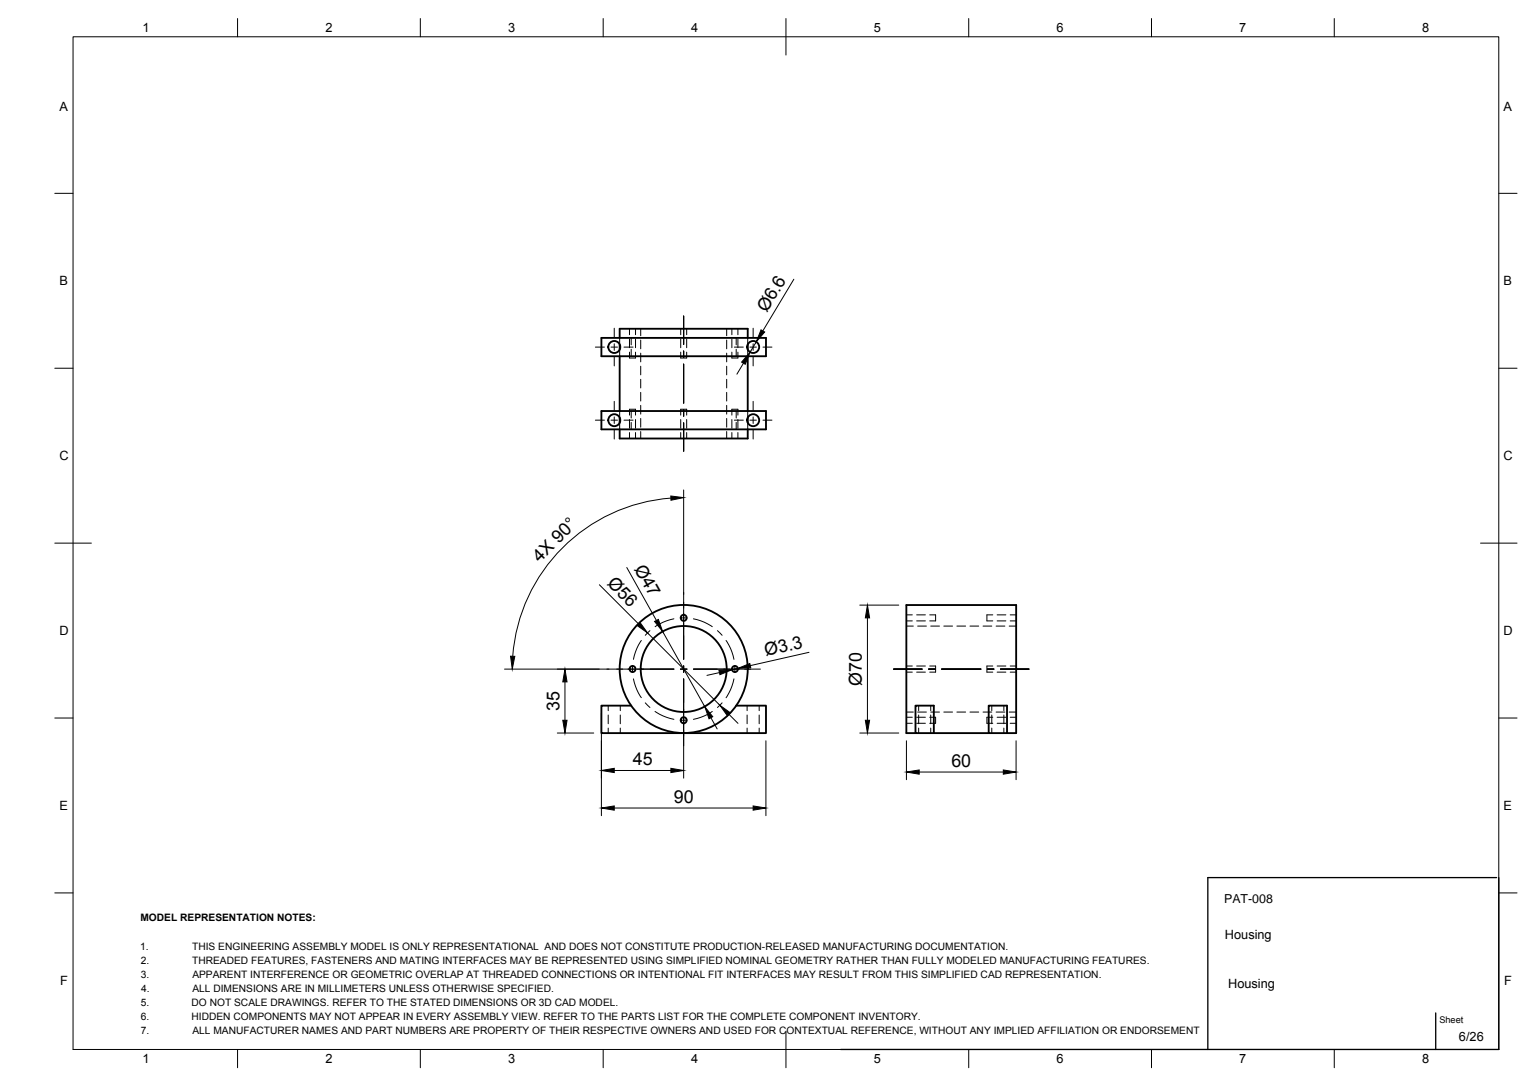
ISO-10303-21;
HEADER;
/* Generated by software containing ST-Developer
 * from STEP Tools, Inc. (www.steptools.com) 
 */

FILE_DESCRIPTION(
/* description */ ('Bearing housing with oil seal and end cap'),
/* implementation_level */ '2;1');

FILE_NAME(
/* name */ 'Housing.step',
/* time_stamp */ '2026-10-28T03:23:10-07:00',
/* author */ (''),
/* organization */ (''),
/* preprocessor_version */ 'ST-DEVELOPER v20.2',
/* originating_system */ 'Autodesk Translation Framework v15.17.0.0',
/* authorisation */ '');

FILE_SCHEMA (('AUTOMOTIVE_DESIGN { 1 0 10303 214 3 1 1 }'));
ENDSEC;

DATA;
#10=MECHANICAL_DESIGN_GEOMETRIC_PRESENTATION_REPRESENTATION('',(#260),#7871);
#218=SHAPE_REPRESENTATION_RELATIONSHIP('SRR','None',#7965,#239);
#239=ADVANCED_BREP_SHAPE_REPRESENTATION('',(#289),#7849);
#260=STYLED_ITEM('',(#8132),#289);
#289=MANIFOLD_SOLID_BREP('Body1',#4086);
#323=FACE_BOUND('',#846,.T.);
#324=FACE_BOUND('',#848,.T.);
#325=FACE_BOUND('',#851,.T.);
#326=FACE_BOUND('',#852,.T.);
#327=FACE_BOUND('',#859,.T.);
#328=FACE_BOUND('',#861,.T.);
#329=FACE_BOUND('',#864,.T.);
#330=FACE_BOUND('',#865,.T.);
#331=FACE_BOUND('',#869,.T.);
#332=FACE_BOUND('',#870,.T.);
#333=FACE_BOUND('',#872,.T.);
#334=FACE_BOUND('',#873,.T.);
#335=FACE_BOUND('',#874,.T.);
#336=FACE_BOUND('',#875,.T.);
#337=FACE_BOUND('',#876,.T.);
#338=FACE_BOUND('',#878,.T.);
#339=FACE_BOUND('',#879,.T.);
#340=FACE_BOUND('',#880,.T.);
#341=FACE_BOUND('',#881,.T.);
#342=FACE_BOUND('',#882,.T.);
#414=PLANE('',#4373);
#415=PLANE('',#4377);
#416=PLANE('',#4381);
#417=PLANE('',#4385);
#418=PLANE('',#4389);
#419=PLANE('',#4393);
#420=PLANE('',#4397);
#421=PLANE('',#4401);
#422=PLANE('',#4414);
#423=PLANE('',#4416);
#424=PLANE('',#4418);
#425=PLANE('',#4420);
#426=PLANE('',#4422);
#427=PLANE('',#4423);
#428=PLANE('',#4424);
#429=PLANE('',#4425);
#430=PLANE('',#4426);
#431=PLANE('',#4427);
#432=PLANE('',#4429);
#433=PLANE('',#4431);
#434=PLANE('',#4433);
#435=PLANE('',#4435);
#436=PLANE('',#4436);
#437=PLANE('',#4437);
#438=PLANE('',#4438);
#439=PLANE('',#4439);
#440=PLANE('',#4446);
#441=PLANE('',#4447);
#562=FACE_OUTER_BOUND('',#821,.T.);
#563=FACE_OUTER_BOUND('',#822,.T.);
#564=FACE_OUTER_BOUND('',#823,.T.);
#565=FACE_OUTER_BOUND('',#824,.T.);
#566=FACE_OUTER_BOUND('',#825,.T.);
#567=FACE_OUTER_BOUND('',#826,.T.);
#568=FACE_OUTER_BOUND('',#827,.T.);
#569=FACE_OUTER_BOUND('',#828,.T.);
#570=FACE_OUTER_BOUND('',#829,.T.);
#571=FACE_OUTER_BOUND('',#830,.T.);
#572=FACE_OUTER_BOUND('',#831,.T.);
#573=FACE_OUTER_BOUND('',#832,.T.);
#574=FACE_OUTER_BOUND('',#833,.T.);
#575=FACE_OUTER_BOUND('',#834,.T.);
#576=FACE_OUTER_BOUND('',#835,.T.);
#577=FACE_OUTER_BOUND('',#836,.T.);
#578=FACE_OUTER_BOUND('',#837,.T.);
#579=FACE_OUTER_BOUND('',#838,.T.);
#580=FACE_OUTER_BOUND('',#839,.T.);
#581=FACE_OUTER_BOUND('',#840,.T.);
#582=FACE_OUTER_BOUND('',#841,.T.);
#583=FACE_OUTER_BOUND('',#842,.T.);
#584=FACE_OUTER_BOUND('',#843,.T.);
#585=FACE_OUTER_BOUND('',#844,.T.);
#586=FACE_OUTER_BOUND('',#845,.T.);
#587=FACE_OUTER_BOUND('',#847,.T.);
#588=FACE_OUTER_BOUND('',#849,.T.);
#589=FACE_OUTER_BOUND('',#850,.T.);
#590=FACE_OUTER_BOUND('',#853,.T.);
#591=FACE_OUTER_BOUND('',#854,.T.);
#592=FACE_OUTER_BOUND('',#855,.T.);
#593=FACE_OUTER_BOUND('',#856,.T.);
#594=FACE_OUTER_BOUND('',#857,.T.);
#595=FACE_OUTER_BOUND('',#858,.T.);
#596=FACE_OUTER_BOUND('',#860,.T.);
#597=FACE_OUTER_BOUND('',#862,.T.);
#598=FACE_OUTER_BOUND('',#863,.T.);
#599=FACE_OUTER_BOUND('',#866,.T.);
#600=FACE_OUTER_BOUND('',#867,.T.);
#601=FACE_OUTER_BOUND('',#868,.T.);
#602=FACE_OUTER_BOUND('',#871,.T.);
#603=FACE_OUTER_BOUND('',#877,.T.);
#821=EDGE_LOOP('',(#2791,#2792,#2793,#2794));
#822=EDGE_LOOP('',(#2795));
#823=EDGE_LOOP('',(#2796,#2797,#2798,#2799));
#824=EDGE_LOOP('',(#2800));
#825=EDGE_LOOP('',(#2801,#2802,#2803,#2804));
#826=EDGE_LOOP('',(#2805));
#827=EDGE_LOOP('',(#2806,#2807,#2808,#2809));
#828=EDGE_LOOP('',(#2810));
#829=EDGE_LOOP('',(#2811,#2812,#2813,#2814));
#830=EDGE_LOOP('',(#2815));
#831=EDGE_LOOP('',(#2816,#2817,#2818,#2819));
#832=EDGE_LOOP('',(#2820));
#833=EDGE_LOOP('',(#2821,#2822,#2823,#2824));
#834=EDGE_LOOP('',(#2825));
#835=EDGE_LOOP('',(#2826,#2827,#2828,#2829));
#836=EDGE_LOOP('',(#2830));
#837=EDGE_LOOP('',(#2831,#2832,#2833,#2834));
#838=EDGE_LOOP('',(#2835,#2836,#2837,#2838));
#839=EDGE_LOOP('',(#2839,#2840,#2841,#2842));
#840=EDGE_LOOP('',(#2843,#2844,#2845,#2846));
#841=EDGE_LOOP('',(#2847,#2848,#2849,#2850));
#842=EDGE_LOOP('',(#2851,#2852,#2853,#2854));
#843=EDGE_LOOP('',(#2855,#2856,#2857,#2858));
#844=EDGE_LOOP('',(#2859,#2860,#2861,#2862));
#845=EDGE_LOOP('',(#2863,#2864,#2865,#2866));
#846=EDGE_LOOP('',(#2867));
#847=EDGE_LOOP('',(#2868,#2869,#2870,#2871));
#848=EDGE_LOOP('',(#2872));
#849=EDGE_LOOP('',(#2873,#2874,#2875,#2876));
#850=EDGE_LOOP('',(#2877,#2878,#2879,#2880,#2881,#2882));
#851=EDGE_LOOP('',(#2883));
#852=EDGE_LOOP('',(#2884));
#853=EDGE_LOOP('',(#2885,#2886,#2887,#2888));
#854=EDGE_LOOP('',(#2889,#2890,#2891,#2892));
#855=EDGE_LOOP('',(#2893,#2894,#2895,#2896));
#856=EDGE_LOOP('',(#2897,#2898,#2899,#2900));
#857=EDGE_LOOP('',(#2901,#2902,#2903,#2904));
#858=EDGE_LOOP('',(#2905,#2906,#2907,#2908));
#859=EDGE_LOOP('',(#2909));
#860=EDGE_LOOP('',(#2910,#2911,#2912,#2913));
#861=EDGE_LOOP('',(#2914));
#862=EDGE_LOOP('',(#2915,#2916,#2917,#2918));
#863=EDGE_LOOP('',(#2919,#2920,#2921,#2922,#2923,#2924));
#864=EDGE_LOOP('',(#2925));
#865=EDGE_LOOP('',(#2926));
#866=EDGE_LOOP('',(#2927,#2928,#2929,#2930));
#867=EDGE_LOOP('',(#2931,#2932,#2933,#2934));
#868=EDGE_LOOP('',(#2935,#2936,#2937,#2938));
#869=EDGE_LOOP('',(#2939,#2940,#2941,#2942,#2943,#2944));
#870=EDGE_LOOP('',(#2945,#2946,#2947,#2948,#2949,#2950));
#871=EDGE_LOOP('',(#2951));
#872=EDGE_LOOP('',(#2952));
#873=EDGE_LOOP('',(#2953));
#874=EDGE_LOOP('',(#2954));
#875=EDGE_LOOP('',(#2955));
#876=EDGE_LOOP('',(#2956));
#877=EDGE_LOOP('',(#2957));
#878=EDGE_LOOP('',(#2958));
#879=EDGE_LOOP('',(#2959));
#880=EDGE_LOOP('',(#2960));
#881=EDGE_LOOP('',(#2961));
#882=EDGE_LOOP('',(#2962));
#1163=LINE('',#6264,#1425);
#1164=LINE('',#6271,#1426);
#1165=LINE('',#6278,#1427);
#1166=LINE('',#6285,#1428);
#1167=LINE('',#6292,#1429);
#1168=LINE('',#6299,#1430);
#1169=LINE('',#6306,#1431);
#1170=LINE('',#6313,#1432);
#1171=LINE('',#6320,#1433);
#1172=LINE('',#6326,#1434);
#1173=LINE('',#6332,#1435);
#1174=LINE('',#6338,#1436);
#1175=LINE('',#6345,#1437);
#1176=LINE('',#6347,#1438);
#1177=LINE('',#6348,#1439);
#1178=LINE('',#6353,#1440);
#1179=LINE('',#6355,#1441);
#1180=LINE('',#6356,#1442);
#1181=LINE('',#6362,#1443);
#1182=LINE('',#6364,#1444);
#1183=LINE('',#6365,#1445);
#1184=LINE('',#6370,#1446);
#1185=LINE('',#6372,#1447);
#1186=LINE('',#6373,#1448);
#1187=LINE('',#6375,#1449);
#1188=LINE('',#6376,#1450);
#1189=LINE('',#6378,#1451);
#1190=LINE('',#6379,#1452);
#1191=LINE('',#6381,#1453);
#1192=LINE('',#6383,#1454);
#1193=LINE('',#6390,#1455);
#1194=LINE('',#6392,#1456);
#1195=LINE('',#6393,#1457);
#1196=LINE('',#6398,#1458);
#1197=LINE('',#6400,#1459);
#1198=LINE('',#6401,#1460);
#1199=LINE('',#6407,#1461);
#1200=LINE('',#6409,#1462);
#1201=LINE('',#6410,#1463);
#1202=LINE('',#6415,#1464);
#1203=LINE('',#6417,#1465);
#1204=LINE('',#6418,#1466);
#1205=LINE('',#6420,#1467);
#1206=LINE('',#6421,#1468);
#1207=LINE('',#6423,#1469);
#1208=LINE('',#6424,#1470);
#1209=LINE('',#6426,#1471);
#1210=LINE('',#6428,#1472);
#1211=LINE('',#6434,#1473);
#1212=LINE('',#6440,#1474);
#1425=VECTOR('',#4944,0.165);
#1426=VECTOR('',#4953,0.165);
#1427=VECTOR('',#4962,0.165);
#1428=VECTOR('',#4971,0.165);
#1429=VECTOR('',#4980,0.165);
#1430=VECTOR('',#4989,0.165);
#1431=VECTOR('',#4998,0.165);
#1432=VECTOR('',#5007,0.165);
#1433=VECTOR('',#5016,0.33);
#1434=VECTOR('',#5023,0.33);
#1435=VECTOR('',#5030,0.33);
#1436=VECTOR('',#5037,0.33);
#1437=VECTOR('',#5044,1.);
#1438=VECTOR('',#5045,1.);
#1439=VECTOR('',#5046,1.);
#1440=VECTOR('',#5051,1.);
#1441=VECTOR('',#5052,1.);
#1442=VECTOR('',#5053,1.);
#1443=VECTOR('',#5058,1.);
#1444=VECTOR('',#5059,1.);
#1445=VECTOR('',#5060,1.);
#1446=VECTOR('',#5065,1.);
#1447=VECTOR('',#5066,1.);
#1448=VECTOR('',#5067,1.);
#1449=VECTOR('',#5070,1.);
#1450=VECTOR('',#5071,1.);
#1451=VECTOR('',#5074,1.);
#1452=VECTOR('',#5075,1.);
#1453=VECTOR('',#5078,1.);
#1454=VECTOR('',#5081,1.);
#1455=VECTOR('',#5088,1.);
#1456=VECTOR('',#5089,1.);
#1457=VECTOR('',#5090,1.);
#1458=VECTOR('',#5095,1.);
#1459=VECTOR('',#5096,1.);
#1460=VECTOR('',#5097,1.);
#1461=VECTOR('',#5102,1.);
#1462=VECTOR('',#5103,1.);
#1463=VECTOR('',#5104,1.);
#1464=VECTOR('',#5109,1.);
#1465=VECTOR('',#5110,1.);
#1466=VECTOR('',#5111,1.);
#1467=VECTOR('',#5114,1.);
#1468=VECTOR('',#5115,1.);
#1469=VECTOR('',#5118,1.);
#1470=VECTOR('',#5119,1.);
#1471=VECTOR('',#5122,1.);
#1472=VECTOR('',#5125,1.);
#1473=VECTOR('',#5132,2.35);
#1474=VECTOR('',#5139,3.5);
#1679=CIRCLE('',#4371,0.165);
#1680=CIRCLE('',#4372,0.165);
#1681=CIRCLE('',#4375,0.165);
#1682=CIRCLE('',#4376,0.165);
#1683=CIRCLE('',#4379,0.165);
#1684=CIRCLE('',#4380,0.165);
#1685=CIRCLE('',#4383,0.165);
#1686=CIRCLE('',#4384,0.165);
#1687=CIRCLE('',#4387,0.165);
#1688=CIRCLE('',#4388,0.165);
#1689=CIRCLE('',#4391,0.165);
#1690=CIRCLE('',#4392,0.165);
#1691=CIRCLE('',#4395,0.165);
#1692=CIRCLE('',#4396,0.165);
#1693=CIRCLE('',#4399,0.165);
#1694=CIRCLE('',#4400,0.165);
#1695=CIRCLE('',#4403,0.33);
#1696=CIRCLE('',#4404,0.33);
#1697=CIRCLE('',#4406,0.33);
#1698=CIRCLE('',#4407,0.33);
#1699=CIRCLE('',#4409,0.33);
#1700=CIRCLE('',#4410,0.33);
#1701=CIRCLE('',#4412,0.33);
#1702=CIRCLE('',#4413,0.33);
#1703=CIRCLE('',#4415,3.5);
#1704=CIRCLE('',#4417,3.5);
#1705=CIRCLE('',#4419,3.5);
#1706=CIRCLE('',#4421,3.5);
#1707=CIRCLE('',#4428,3.5);
#1708=CIRCLE('',#4430,3.5);
#1709=CIRCLE('',#4432,3.5);
#1710=CIRCLE('',#4434,3.5);
#1711=CIRCLE('',#4441,2.35);
#1712=CIRCLE('',#4442,2.35);
#1713=CIRCLE('',#4444,3.5);
#1714=CIRCLE('',#4445,3.5);
#1907=VERTEX_POINT('',#6261);
#1908=VERTEX_POINT('',#6263);
#1909=VERTEX_POINT('',#6268);
#1910=VERTEX_POINT('',#6270);
#1911=VERTEX_POINT('',#6275);
#1912=VERTEX_POINT('',#6277);
#1913=VERTEX_POINT('',#6282);
#1914=VERTEX_POINT('',#6284);
#1915=VERTEX_POINT('',#6289);
#1916=VERTEX_POINT('',#6291);
#1917=VERTEX_POINT('',#6296);
#1918=VERTEX_POINT('',#6298);
#1919=VERTEX_POINT('',#6303);
#1920=VERTEX_POINT('',#6305);
#1921=VERTEX_POINT('',#6310);
#1922=VERTEX_POINT('',#6312);
#1923=VERTEX_POINT('',#6317);
#1924=VERTEX_POINT('',#6319);
#1925=VERTEX_POINT('',#6323);
#1926=VERTEX_POINT('',#6325);
#1927=VERTEX_POINT('',#6329);
#1928=VERTEX_POINT('',#6331);
#1929=VERTEX_POINT('',#6335);
#1930=VERTEX_POINT('',#6337);
#1931=VERTEX_POINT('',#6341);
#1932=VERTEX_POINT('',#6342);
#1933=VERTEX_POINT('',#6344);
#1934=VERTEX_POINT('',#6346);
#1935=VERTEX_POINT('',#6350);
#1936=VERTEX_POINT('',#6352);
#1937=VERTEX_POINT('',#6354);
#1938=VERTEX_POINT('',#6358);
#1939=VERTEX_POINT('',#6359);
#1940=VERTEX_POINT('',#6361);
#1941=VERTEX_POINT('',#6363);
#1942=VERTEX_POINT('',#6367);
#1943=VERTEX_POINT('',#6369);
#1944=VERTEX_POINT('',#6371);
#1945=VERTEX_POINT('',#6386);
#1946=VERTEX_POINT('',#6387);
#1947=VERTEX_POINT('',#6389);
#1948=VERTEX_POINT('',#6391);
#1949=VERTEX_POINT('',#6395);
#1950=VERTEX_POINT('',#6397);
#1951=VERTEX_POINT('',#6399);
#1952=VERTEX_POINT('',#6403);
#1953=VERTEX_POINT('',#6404);
#1954=VERTEX_POINT('',#6406);
#1955=VERTEX_POINT('',#6408);
#1956=VERTEX_POINT('',#6412);
#1957=VERTEX_POINT('',#6414);
#1958=VERTEX_POINT('',#6416);
#1959=VERTEX_POINT('',#6431);
#1960=VERTEX_POINT('',#6433);
#1961=VERTEX_POINT('',#6437);
#1962=VERTEX_POINT('',#6439);
#2259=EDGE_CURVE('',#1907,#1907,#1679,.T.);
#2260=EDGE_CURVE('',#1907,#1908,#1163,.T.);
#2261=EDGE_CURVE('',#1908,#1908,#1680,.T.);
#2262=EDGE_CURVE('',#1909,#1909,#1681,.T.);
#2263=EDGE_CURVE('',#1909,#1910,#1164,.T.);
#2264=EDGE_CURVE('',#1910,#1910,#1682,.T.);
#2265=EDGE_CURVE('',#1911,#1911,#1683,.T.);
#2266=EDGE_CURVE('',#1911,#1912,#1165,.T.);
#2267=EDGE_CURVE('',#1912,#1912,#1684,.T.);
#2268=EDGE_CURVE('',#1913,#1913,#1685,.T.);
#2269=EDGE_CURVE('',#1913,#1914,#1166,.T.);
#2270=EDGE_CURVE('',#1914,#1914,#1686,.T.);
#2271=EDGE_CURVE('',#1915,#1915,#1687,.T.);
#2272=EDGE_CURVE('',#1915,#1916,#1167,.T.);
#2273=EDGE_CURVE('',#1916,#1916,#1688,.T.);
#2274=EDGE_CURVE('',#1917,#1917,#1689,.T.);
#2275=EDGE_CURVE('',#1917,#1918,#1168,.T.);
#2276=EDGE_CURVE('',#1918,#1918,#1690,.T.);
#2277=EDGE_CURVE('',#1919,#1919,#1691,.T.);
#2278=EDGE_CURVE('',#1919,#1920,#1169,.T.);
#2279=EDGE_CURVE('',#1920,#1920,#1692,.T.);
#2280=EDGE_CURVE('',#1921,#1921,#1693,.T.);
#2281=EDGE_CURVE('',#1921,#1922,#1170,.T.);
#2282=EDGE_CURVE('',#1922,#1922,#1694,.T.);
#2283=EDGE_CURVE('',#1923,#1923,#1695,.T.);
#2284=EDGE_CURVE('',#1923,#1924,#1171,.T.);
#2285=EDGE_CURVE('',#1924,#1924,#1696,.T.);
#2286=EDGE_CURVE('',#1925,#1925,#1697,.T.);
#2287=EDGE_CURVE('',#1925,#1926,#1172,.T.);
#2288=EDGE_CURVE('',#1926,#1926,#1698,.T.);
#2289=EDGE_CURVE('',#1927,#1927,#1699,.T.);
#2290=EDGE_CURVE('',#1927,#1928,#1173,.T.);
#2291=EDGE_CURVE('',#1928,#1928,#1700,.T.);
#2292=EDGE_CURVE('',#1929,#1929,#1701,.T.);
#2293=EDGE_CURVE('',#1929,#1930,#1174,.T.);
#2294=EDGE_CURVE('',#1930,#1930,#1702,.T.);
#2295=EDGE_CURVE('',#1931,#1932,#1703,.T.);
#2296=EDGE_CURVE('',#1931,#1933,#1175,.T.);
#2297=EDGE_CURVE('',#1933,#1934,#1176,.T.);
#2298=EDGE_CURVE('',#1934,#1932,#1177,.T.);
#2299=EDGE_CURVE('',#1932,#1935,#1704,.T.);
#2300=EDGE_CURVE('',#1932,#1936,#1178,.T.);
#2301=EDGE_CURVE('',#1936,#1937,#1179,.T.);
#2302=EDGE_CURVE('',#1937,#1935,#1180,.T.);
#2303=EDGE_CURVE('',#1938,#1939,#1705,.T.);
#2304=EDGE_CURVE('',#1938,#1940,#1181,.T.);
#2305=EDGE_CURVE('',#1940,#1941,#1182,.T.);
#2306=EDGE_CURVE('',#1941,#1939,#1183,.T.);
#2307=EDGE_CURVE('',#1942,#1938,#1706,.T.);
#2308=EDGE_CURVE('',#1942,#1943,#1184,.T.);
#2309=EDGE_CURVE('',#1943,#1944,#1185,.T.);
#2310=EDGE_CURVE('',#1944,#1938,#1186,.T.);
#2311=EDGE_CURVE('',#1939,#1931,#1187,.T.);
#2312=EDGE_CURVE('',#1941,#1933,#1188,.T.);
#2313=EDGE_CURVE('',#1935,#1942,#1189,.T.);
#2314=EDGE_CURVE('',#1943,#1937,#1190,.T.);
#2315=EDGE_CURVE('',#1944,#1936,#1191,.T.);
#2316=EDGE_CURVE('',#1940,#1934,#1192,.T.);
#2317=EDGE_CURVE('',#1945,#1946,#1707,.T.);
#2318=EDGE_CURVE('',#1945,#1947,#1193,.T.);
#2319=EDGE_CURVE('',#1947,#1948,#1194,.T.);
#2320=EDGE_CURVE('',#1948,#1946,#1195,.T.);
#2321=EDGE_CURVE('',#1946,#1949,#1708,.T.);
#2322=EDGE_CURVE('',#1946,#1950,#1196,.T.);
#2323=EDGE_CURVE('',#1950,#1951,#1197,.T.);
#2324=EDGE_CURVE('',#1951,#1949,#1198,.T.);
#2325=EDGE_CURVE('',#1952,#1953,#1709,.T.);
#2326=EDGE_CURVE('',#1952,#1954,#1199,.T.);
#2327=EDGE_CURVE('',#1954,#1955,#1200,.T.);
#2328=EDGE_CURVE('',#1955,#1953,#1201,.T.);
#2329=EDGE_CURVE('',#1956,#1952,#1710,.T.);
#2330=EDGE_CURVE('',#1956,#1957,#1202,.T.);
#2331=EDGE_CURVE('',#1957,#1958,#1203,.T.);
#2332=EDGE_CURVE('',#1958,#1952,#1204,.T.);
#2333=EDGE_CURVE('',#1953,#1945,#1205,.T.);
#2334=EDGE_CURVE('',#1955,#1947,#1206,.T.);
#2335=EDGE_CURVE('',#1949,#1956,#1207,.T.);
#2336=EDGE_CURVE('',#1957,#1951,#1208,.T.);
#2337=EDGE_CURVE('',#1958,#1950,#1209,.T.);
#2338=EDGE_CURVE('',#1954,#1948,#1210,.T.);
#2339=EDGE_CURVE('',#1959,#1959,#1711,.T.);
#2340=EDGE_CURVE('',#1959,#1960,#1211,.T.);
#2341=EDGE_CURVE('',#1960,#1960,#1712,.T.);
#2342=EDGE_CURVE('',#1961,#1961,#1713,.T.);
#2343=EDGE_CURVE('',#1961,#1962,#1212,.T.);
#2344=EDGE_CURVE('',#1962,#1962,#1714,.T.);
#2791=ORIENTED_EDGE('',*,*,#2259,.F.);
#2792=ORIENTED_EDGE('',*,*,#2260,.T.);
#2793=ORIENTED_EDGE('',*,*,#2261,.F.);
#2794=ORIENTED_EDGE('',*,*,#2260,.F.);
#2795=ORIENTED_EDGE('',*,*,#2259,.T.);
#2796=ORIENTED_EDGE('',*,*,#2262,.F.);
#2797=ORIENTED_EDGE('',*,*,#2263,.T.);
#2798=ORIENTED_EDGE('',*,*,#2264,.F.);
#2799=ORIENTED_EDGE('',*,*,#2263,.F.);
#2800=ORIENTED_EDGE('',*,*,#2262,.T.);
#2801=ORIENTED_EDGE('',*,*,#2265,.F.);
#2802=ORIENTED_EDGE('',*,*,#2266,.T.);
#2803=ORIENTED_EDGE('',*,*,#2267,.F.);
#2804=ORIENTED_EDGE('',*,*,#2266,.F.);
#2805=ORIENTED_EDGE('',*,*,#2265,.T.);
#2806=ORIENTED_EDGE('',*,*,#2268,.F.);
#2807=ORIENTED_EDGE('',*,*,#2269,.T.);
#2808=ORIENTED_EDGE('',*,*,#2270,.F.);
#2809=ORIENTED_EDGE('',*,*,#2269,.F.);
#2810=ORIENTED_EDGE('',*,*,#2268,.T.);
#2811=ORIENTED_EDGE('',*,*,#2271,.F.);
#2812=ORIENTED_EDGE('',*,*,#2272,.T.);
#2813=ORIENTED_EDGE('',*,*,#2273,.T.);
#2814=ORIENTED_EDGE('',*,*,#2272,.F.);
#2815=ORIENTED_EDGE('',*,*,#2273,.F.);
#2816=ORIENTED_EDGE('',*,*,#2274,.F.);
#2817=ORIENTED_EDGE('',*,*,#2275,.T.);
#2818=ORIENTED_EDGE('',*,*,#2276,.T.);
#2819=ORIENTED_EDGE('',*,*,#2275,.F.);
#2820=ORIENTED_EDGE('',*,*,#2276,.F.);
#2821=ORIENTED_EDGE('',*,*,#2277,.F.);
#2822=ORIENTED_EDGE('',*,*,#2278,.T.);
#2823=ORIENTED_EDGE('',*,*,#2279,.T.);
#2824=ORIENTED_EDGE('',*,*,#2278,.F.);
#2825=ORIENTED_EDGE('',*,*,#2279,.F.);
#2826=ORIENTED_EDGE('',*,*,#2280,.F.);
#2827=ORIENTED_EDGE('',*,*,#2281,.T.);
#2828=ORIENTED_EDGE('',*,*,#2282,.T.);
#2829=ORIENTED_EDGE('',*,*,#2281,.F.);
#2830=ORIENTED_EDGE('',*,*,#2282,.F.);
#2831=ORIENTED_EDGE('',*,*,#2283,.F.);
#2832=ORIENTED_EDGE('',*,*,#2284,.T.);
#2833=ORIENTED_EDGE('',*,*,#2285,.F.);
#2834=ORIENTED_EDGE('',*,*,#2284,.F.);
#2835=ORIENTED_EDGE('',*,*,#2286,.F.);
#2836=ORIENTED_EDGE('',*,*,#2287,.T.);
#2837=ORIENTED_EDGE('',*,*,#2288,.F.);
#2838=ORIENTED_EDGE('',*,*,#2287,.F.);
#2839=ORIENTED_EDGE('',*,*,#2289,.F.);
#2840=ORIENTED_EDGE('',*,*,#2290,.T.);
#2841=ORIENTED_EDGE('',*,*,#2291,.F.);
#2842=ORIENTED_EDGE('',*,*,#2290,.F.);
#2843=ORIENTED_EDGE('',*,*,#2292,.F.);
#2844=ORIENTED_EDGE('',*,*,#2293,.T.);
#2845=ORIENTED_EDGE('',*,*,#2294,.F.);
#2846=ORIENTED_EDGE('',*,*,#2293,.F.);
#2847=ORIENTED_EDGE('',*,*,#2295,.F.);
#2848=ORIENTED_EDGE('',*,*,#2296,.T.);
#2849=ORIENTED_EDGE('',*,*,#2297,.T.);
#2850=ORIENTED_EDGE('',*,*,#2298,.T.);
#2851=ORIENTED_EDGE('',*,*,#2299,.F.);
#2852=ORIENTED_EDGE('',*,*,#2300,.T.);
#2853=ORIENTED_EDGE('',*,*,#2301,.T.);
#2854=ORIENTED_EDGE('',*,*,#2302,.T.);
#2855=ORIENTED_EDGE('',*,*,#2303,.F.);
#2856=ORIENTED_EDGE('',*,*,#2304,.T.);
#2857=ORIENTED_EDGE('',*,*,#2305,.T.);
#2858=ORIENTED_EDGE('',*,*,#2306,.T.);
#2859=ORIENTED_EDGE('',*,*,#2307,.F.);
#2860=ORIENTED_EDGE('',*,*,#2308,.T.);
#2861=ORIENTED_EDGE('',*,*,#2309,.T.);
#2862=ORIENTED_EDGE('',*,*,#2310,.T.);
#2863=ORIENTED_EDGE('',*,*,#2311,.F.);
#2864=ORIENTED_EDGE('',*,*,#2306,.F.);
#2865=ORIENTED_EDGE('',*,*,#2312,.T.);
#2866=ORIENTED_EDGE('',*,*,#2296,.F.);
#2867=ORIENTED_EDGE('',*,*,#2294,.T.);
#2868=ORIENTED_EDGE('',*,*,#2313,.F.);
#2869=ORIENTED_EDGE('',*,*,#2302,.F.);
#2870=ORIENTED_EDGE('',*,*,#2314,.F.);
#2871=ORIENTED_EDGE('',*,*,#2308,.F.);
#2872=ORIENTED_EDGE('',*,*,#2288,.T.);
#2873=ORIENTED_EDGE('',*,*,#2309,.F.);
#2874=ORIENTED_EDGE('',*,*,#2314,.T.);
#2875=ORIENTED_EDGE('',*,*,#2301,.F.);
#2876=ORIENTED_EDGE('',*,*,#2315,.F.);
#2877=ORIENTED_EDGE('',*,*,#2298,.F.);
#2878=ORIENTED_EDGE('',*,*,#2316,.F.);
#2879=ORIENTED_EDGE('',*,*,#2304,.F.);
#2880=ORIENTED_EDGE('',*,*,#2310,.F.);
#2881=ORIENTED_EDGE('',*,*,#2315,.T.);
#2882=ORIENTED_EDGE('',*,*,#2300,.F.);
#2883=ORIENTED_EDGE('',*,*,#2286,.T.);
#2884=ORIENTED_EDGE('',*,*,#2292,.T.);
#2885=ORIENTED_EDGE('',*,*,#2305,.F.);
#2886=ORIENTED_EDGE('',*,*,#2316,.T.);
#2887=ORIENTED_EDGE('',*,*,#2297,.F.);
#2888=ORIENTED_EDGE('',*,*,#2312,.F.);
#2889=ORIENTED_EDGE('',*,*,#2317,.F.);
#2890=ORIENTED_EDGE('',*,*,#2318,.T.);
#2891=ORIENTED_EDGE('',*,*,#2319,.T.);
#2892=ORIENTED_EDGE('',*,*,#2320,.T.);
#2893=ORIENTED_EDGE('',*,*,#2321,.F.);
#2894=ORIENTED_EDGE('',*,*,#2322,.T.);
#2895=ORIENTED_EDGE('',*,*,#2323,.T.);
#2896=ORIENTED_EDGE('',*,*,#2324,.T.);
#2897=ORIENTED_EDGE('',*,*,#2325,.F.);
#2898=ORIENTED_EDGE('',*,*,#2326,.T.);
#2899=ORIENTED_EDGE('',*,*,#2327,.T.);
#2900=ORIENTED_EDGE('',*,*,#2328,.T.);
#2901=ORIENTED_EDGE('',*,*,#2329,.F.);
#2902=ORIENTED_EDGE('',*,*,#2330,.T.);
#2903=ORIENTED_EDGE('',*,*,#2331,.T.);
#2904=ORIENTED_EDGE('',*,*,#2332,.T.);
#2905=ORIENTED_EDGE('',*,*,#2333,.F.);
#2906=ORIENTED_EDGE('',*,*,#2328,.F.);
#2907=ORIENTED_EDGE('',*,*,#2334,.T.);
#2908=ORIENTED_EDGE('',*,*,#2318,.F.);
#2909=ORIENTED_EDGE('',*,*,#2285,.T.);
#2910=ORIENTED_EDGE('',*,*,#2335,.F.);
#2911=ORIENTED_EDGE('',*,*,#2324,.F.);
#2912=ORIENTED_EDGE('',*,*,#2336,.F.);
#2913=ORIENTED_EDGE('',*,*,#2330,.F.);
#2914=ORIENTED_EDGE('',*,*,#2291,.T.);
#2915=ORIENTED_EDGE('',*,*,#2331,.F.);
#2916=ORIENTED_EDGE('',*,*,#2336,.T.);
#2917=ORIENTED_EDGE('',*,*,#2323,.F.);
#2918=ORIENTED_EDGE('',*,*,#2337,.F.);
#2919=ORIENTED_EDGE('',*,*,#2320,.F.);
#2920=ORIENTED_EDGE('',*,*,#2338,.F.);
#2921=ORIENTED_EDGE('',*,*,#2326,.F.);
#2922=ORIENTED_EDGE('',*,*,#2332,.F.);
#2923=ORIENTED_EDGE('',*,*,#2337,.T.);
#2924=ORIENTED_EDGE('',*,*,#2322,.F.);
#2925=ORIENTED_EDGE('',*,*,#2283,.T.);
#2926=ORIENTED_EDGE('',*,*,#2289,.T.);
#2927=ORIENTED_EDGE('',*,*,#2327,.F.);
#2928=ORIENTED_EDGE('',*,*,#2338,.T.);
#2929=ORIENTED_EDGE('',*,*,#2319,.F.);
#2930=ORIENTED_EDGE('',*,*,#2334,.F.);
#2931=ORIENTED_EDGE('',*,*,#2339,.F.);
#2932=ORIENTED_EDGE('',*,*,#2340,.T.);
#2933=ORIENTED_EDGE('',*,*,#2341,.T.);
#2934=ORIENTED_EDGE('',*,*,#2340,.F.);
#2935=ORIENTED_EDGE('',*,*,#2342,.F.);
#2936=ORIENTED_EDGE('',*,*,#2343,.T.);
#2937=ORIENTED_EDGE('',*,*,#2344,.T.);
#2938=ORIENTED_EDGE('',*,*,#2343,.F.);
#2939=ORIENTED_EDGE('',*,*,#2311,.T.);
#2940=ORIENTED_EDGE('',*,*,#2295,.T.);
#2941=ORIENTED_EDGE('',*,*,#2299,.T.);
#2942=ORIENTED_EDGE('',*,*,#2313,.T.);
#2943=ORIENTED_EDGE('',*,*,#2307,.T.);
#2944=ORIENTED_EDGE('',*,*,#2303,.T.);
#2945=ORIENTED_EDGE('',*,*,#2333,.T.);
#2946=ORIENTED_EDGE('',*,*,#2317,.T.);
#2947=ORIENTED_EDGE('',*,*,#2321,.T.);
#2948=ORIENTED_EDGE('',*,*,#2335,.T.);
#2949=ORIENTED_EDGE('',*,*,#2329,.T.);
#2950=ORIENTED_EDGE('',*,*,#2325,.T.);
#2951=ORIENTED_EDGE('',*,*,#2342,.T.);
#2952=ORIENTED_EDGE('',*,*,#2339,.T.);
#2953=ORIENTED_EDGE('',*,*,#2270,.T.);
#2954=ORIENTED_EDGE('',*,*,#2267,.T.);
#2955=ORIENTED_EDGE('',*,*,#2264,.T.);
#2956=ORIENTED_EDGE('',*,*,#2261,.T.);
#2957=ORIENTED_EDGE('',*,*,#2344,.F.);
#2958=ORIENTED_EDGE('',*,*,#2341,.F.);
#2959=ORIENTED_EDGE('',*,*,#2280,.T.);
#2960=ORIENTED_EDGE('',*,*,#2277,.T.);
#2961=ORIENTED_EDGE('',*,*,#2274,.T.);
#2962=ORIENTED_EDGE('',*,*,#2271,.T.);
#3763=CYLINDRICAL_SURFACE('',#4370,0.165);
#3764=CYLINDRICAL_SURFACE('',#4374,0.165);
#3765=CYLINDRICAL_SURFACE('',#4378,0.165);
#3766=CYLINDRICAL_SURFACE('',#4382,0.165);
#3767=CYLINDRICAL_SURFACE('',#4386,0.165);
#3768=CYLINDRICAL_SURFACE('',#4390,0.165);
#3769=CYLINDRICAL_SURFACE('',#4394,0.165);
#3770=CYLINDRICAL_SURFACE('',#4398,0.165);
#3771=CYLINDRICAL_SURFACE('',#4402,0.33);
#3772=CYLINDRICAL_SURFACE('',#4405,0.33);
#3773=CYLINDRICAL_SURFACE('',#4408,0.33);
#3774=CYLINDRICAL_SURFACE('',#4411,0.33);
#3775=CYLINDRICAL_SURFACE('',#4440,2.35);
#3776=CYLINDRICAL_SURFACE('',#4443,3.5);
#3844=ADVANCED_FACE('',(#562),#3763,.F.);
#3845=ADVANCED_FACE('',(#563),#414,.T.);
#3846=ADVANCED_FACE('',(#564),#3764,.F.);
#3847=ADVANCED_FACE('',(#565),#415,.T.);
#3848=ADVANCED_FACE('',(#566),#3765,.F.);
#3849=ADVANCED_FACE('',(#567),#416,.T.);
#3850=ADVANCED_FACE('',(#568),#3766,.F.);
#3851=ADVANCED_FACE('',(#569),#417,.T.);
#3852=ADVANCED_FACE('',(#570),#3767,.F.);
#3853=ADVANCED_FACE('',(#571),#418,.F.);
#3854=ADVANCED_FACE('',(#572),#3768,.F.);
#3855=ADVANCED_FACE('',(#573),#419,.F.);
#3856=ADVANCED_FACE('',(#574),#3769,.F.);
#3857=ADVANCED_FACE('',(#575),#420,.F.);
#3858=ADVANCED_FACE('',(#576),#3770,.F.);
#3859=ADVANCED_FACE('',(#577),#421,.F.);
#3860=ADVANCED_FACE('',(#578),#3771,.F.);
#3861=ADVANCED_FACE('',(#579),#3772,.F.);
#3862=ADVANCED_FACE('',(#580),#3773,.F.);
#3863=ADVANCED_FACE('',(#581),#3774,.F.);
#3864=ADVANCED_FACE('',(#582),#422,.T.);
#3865=ADVANCED_FACE('',(#583),#423,.T.);
#3866=ADVANCED_FACE('',(#584),#424,.F.);
#3867=ADVANCED_FACE('',(#585),#425,.F.);
#3868=ADVANCED_FACE('',(#586,#323),#426,.T.);
#3869=ADVANCED_FACE('',(#587,#324),#427,.T.);
#3870=ADVANCED_FACE('',(#588),#428,.T.);
#3871=ADVANCED_FACE('',(#589,#325,#326),#429,.T.);
#3872=ADVANCED_FACE('',(#590),#430,.T.);
#3873=ADVANCED_FACE('',(#591),#431,.T.);
#3874=ADVANCED_FACE('',(#592),#432,.T.);
#3875=ADVANCED_FACE('',(#593),#433,.F.);
#3876=ADVANCED_FACE('',(#594),#434,.F.);
#3877=ADVANCED_FACE('',(#595,#327),#435,.T.);
#3878=ADVANCED_FACE('',(#596,#328),#436,.T.);
#3879=ADVANCED_FACE('',(#597),#437,.T.);
#3880=ADVANCED_FACE('',(#598,#329,#330),#438,.T.);
#3881=ADVANCED_FACE('',(#599),#439,.T.);
#3882=ADVANCED_FACE('',(#600),#3775,.F.);
#3883=ADVANCED_FACE('',(#601,#331,#332),#3776,.T.);
#3884=ADVANCED_FACE('',(#602,#333,#334,#335,#336,#337),#440,.T.);
#3885=ADVANCED_FACE('',(#603,#338,#339,#340,#341,#342),#441,.F.);
#4086=CLOSED_SHELL('',(#3844,#3845,#3846,#3847,#3848,#3849,#3850,#3851,
#3852,#3853,#3854,#3855,#3856,#3857,#3858,#3859,#3860,#3861,#3862,#3863,
#3864,#3865,#3866,#3867,#3868,#3869,#3870,#3871,#3872,#3873,#3874,#3875,
#3876,#3877,#3878,#3879,#3880,#3881,#3882,#3883,#3884,#3885));
#4369=AXIS2_PLACEMENT_3D('',#6259,#4938,#4939);
#4370=AXIS2_PLACEMENT_3D('',#6260,#4940,#4941);
#4371=AXIS2_PLACEMENT_3D('',#6262,#4942,#4943);
#4372=AXIS2_PLACEMENT_3D('',#6265,#4945,#4946);
#4373=AXIS2_PLACEMENT_3D('',#6266,#4947,#4948);
#4374=AXIS2_PLACEMENT_3D('',#6267,#4949,#4950);
#4375=AXIS2_PLACEMENT_3D('',#6269,#4951,#4952);
#4376=AXIS2_PLACEMENT_3D('',#6272,#4954,#4955);
#4377=AXIS2_PLACEMENT_3D('',#6273,#4956,#4957);
#4378=AXIS2_PLACEMENT_3D('',#6274,#4958,#4959);
#4379=AXIS2_PLACEMENT_3D('',#6276,#4960,#4961);
#4380=AXIS2_PLACEMENT_3D('',#6279,#4963,#4964);
#4381=AXIS2_PLACEMENT_3D('',#6280,#4965,#4966);
#4382=AXIS2_PLACEMENT_3D('',#6281,#4967,#4968);
#4383=AXIS2_PLACEMENT_3D('',#6283,#4969,#4970);
#4384=AXIS2_PLACEMENT_3D('',#6286,#4972,#4973);
#4385=AXIS2_PLACEMENT_3D('',#6287,#4974,#4975);
#4386=AXIS2_PLACEMENT_3D('',#6288,#4976,#4977);
#4387=AXIS2_PLACEMENT_3D('',#6290,#4978,#4979);
#4388=AXIS2_PLACEMENT_3D('',#6293,#4981,#4982);
#4389=AXIS2_PLACEMENT_3D('',#6294,#4983,#4984);
#4390=AXIS2_PLACEMENT_3D('',#6295,#4985,#4986);
#4391=AXIS2_PLACEMENT_3D('',#6297,#4987,#4988);
#4392=AXIS2_PLACEMENT_3D('',#6300,#4990,#4991);
#4393=AXIS2_PLACEMENT_3D('',#6301,#4992,#4993);
#4394=AXIS2_PLACEMENT_3D('',#6302,#4994,#4995);
#4395=AXIS2_PLACEMENT_3D('',#6304,#4996,#4997);
#4396=AXIS2_PLACEMENT_3D('',#6307,#4999,#5000);
#4397=AXIS2_PLACEMENT_3D('',#6308,#5001,#5002);
#4398=AXIS2_PLACEMENT_3D('',#6309,#5003,#5004);
#4399=AXIS2_PLACEMENT_3D('',#6311,#5005,#5006);
#4400=AXIS2_PLACEMENT_3D('',#6314,#5008,#5009);
#4401=AXIS2_PLACEMENT_3D('',#6315,#5010,#5011);
#4402=AXIS2_PLACEMENT_3D('',#6316,#5012,#5013);
#4403=AXIS2_PLACEMENT_3D('',#6318,#5014,#5015);
#4404=AXIS2_PLACEMENT_3D('',#6321,#5017,#5018);
#4405=AXIS2_PLACEMENT_3D('',#6322,#5019,#5020);
#4406=AXIS2_PLACEMENT_3D('',#6324,#5021,#5022);
#4407=AXIS2_PLACEMENT_3D('',#6327,#5024,#5025);
#4408=AXIS2_PLACEMENT_3D('',#6328,#5026,#5027);
#4409=AXIS2_PLACEMENT_3D('',#6330,#5028,#5029);
#4410=AXIS2_PLACEMENT_3D('',#6333,#5031,#5032);
#4411=AXIS2_PLACEMENT_3D('',#6334,#5033,#5034);
#4412=AXIS2_PLACEMENT_3D('',#6336,#5035,#5036);
#4413=AXIS2_PLACEMENT_3D('',#6339,#5038,#5039);
#4414=AXIS2_PLACEMENT_3D('',#6340,#5040,#5041);
#4415=AXIS2_PLACEMENT_3D('',#6343,#5042,#5043);
#4416=AXIS2_PLACEMENT_3D('',#6349,#5047,#5048);
#4417=AXIS2_PLACEMENT_3D('',#6351,#5049,#5050);
#4418=AXIS2_PLACEMENT_3D('',#6357,#5054,#5055);
#4419=AXIS2_PLACEMENT_3D('',#6360,#5056,#5057);
#4420=AXIS2_PLACEMENT_3D('',#6366,#5061,#5062);
#4421=AXIS2_PLACEMENT_3D('',#6368,#5063,#5064);
#4422=AXIS2_PLACEMENT_3D('',#6374,#5068,#5069);
#4423=AXIS2_PLACEMENT_3D('',#6377,#5072,#5073);
#4424=AXIS2_PLACEMENT_3D('',#6380,#5076,#5077);
#4425=AXIS2_PLACEMENT_3D('',#6382,#5079,#5080);
#4426=AXIS2_PLACEMENT_3D('',#6384,#5082,#5083);
#4427=AXIS2_PLACEMENT_3D('',#6385,#5084,#5085);
#4428=AXIS2_PLACEMENT_3D('',#6388,#5086,#5087);
#4429=AXIS2_PLACEMENT_3D('',#6394,#5091,#5092);
#4430=AXIS2_PLACEMENT_3D('',#6396,#5093,#5094);
#4431=AXIS2_PLACEMENT_3D('',#6402,#5098,#5099);
#4432=AXIS2_PLACEMENT_3D('',#6405,#5100,#5101);
#4433=AXIS2_PLACEMENT_3D('',#6411,#5105,#5106);
#4434=AXIS2_PLACEMENT_3D('',#6413,#5107,#5108);
#4435=AXIS2_PLACEMENT_3D('',#6419,#5112,#5113);
#4436=AXIS2_PLACEMENT_3D('',#6422,#5116,#5117);
#4437=AXIS2_PLACEMENT_3D('',#6425,#5120,#5121);
#4438=AXIS2_PLACEMENT_3D('',#6427,#5123,#5124);
#4439=AXIS2_PLACEMENT_3D('',#6429,#5126,#5127);
#4440=AXIS2_PLACEMENT_3D('',#6430,#5128,#5129);
#4441=AXIS2_PLACEMENT_3D('',#6432,#5130,#5131);
#4442=AXIS2_PLACEMENT_3D('',#6435,#5133,#5134);
#4443=AXIS2_PLACEMENT_3D('',#6436,#5135,#5136);
#4444=AXIS2_PLACEMENT_3D('',#6438,#5137,#5138);
#4445=AXIS2_PLACEMENT_3D('',#6441,#5140,#5141);
#4446=AXIS2_PLACEMENT_3D('',#6442,#5142,#5143);
#4447=AXIS2_PLACEMENT_3D('',#6443,#5144,#5145);
#4938=DIRECTION('axis',(0.,0.,1.));
#4939=DIRECTION('refdir',(1.,0.,0.));
#4940=DIRECTION('center_axis',(0.,1.,0.));
#4941=DIRECTION('ref_axis',(1.,0.,0.));
#4942=DIRECTION('center_axis',(0.,1.,0.));
#4943=DIRECTION('ref_axis',(1.,0.,0.));
#4944=DIRECTION('',(0.,1.,0.));
#4945=DIRECTION('center_axis',(0.,-1.,0.));
#4946=DIRECTION('ref_axis',(1.,0.,0.));
#4947=DIRECTION('center_axis',(0.,1.,0.));
#4948=DIRECTION('ref_axis',(1.,0.,0.));
#4949=DIRECTION('center_axis',(0.,1.,0.));
#4950=DIRECTION('ref_axis',(1.,0.,0.));
#4951=DIRECTION('center_axis',(0.,1.,0.));
#4952=DIRECTION('ref_axis',(1.,0.,0.));
#4953=DIRECTION('',(0.,1.,0.));
#4954=DIRECTION('center_axis',(0.,-1.,0.));
#4955=DIRECTION('ref_axis',(1.,0.,0.));
#4956=DIRECTION('center_axis',(0.,1.,0.));
#4957=DIRECTION('ref_axis',(1.,0.,0.));
#4958=DIRECTION('center_axis',(0.,1.,0.));
#4959=DIRECTION('ref_axis',(1.,0.,0.));
#4960=DIRECTION('center_axis',(0.,1.,0.));
#4961=DIRECTION('ref_axis',(1.,0.,0.));
#4962=DIRECTION('',(0.,1.,0.));
#4963=DIRECTION('center_axis',(0.,-1.,0.));
#4964=DIRECTION('ref_axis',(1.,0.,0.));
#4965=DIRECTION('center_axis',(0.,1.,0.));
#4966=DIRECTION('ref_axis',(1.,0.,0.));
#4967=DIRECTION('center_axis',(0.,1.,0.));
#4968=DIRECTION('ref_axis',(1.,0.,0.));
#4969=DIRECTION('center_axis',(0.,1.,0.));
#4970=DIRECTION('ref_axis',(1.,0.,0.));
#4971=DIRECTION('',(0.,1.,0.));
#4972=DIRECTION('center_axis',(0.,-1.,0.));
#4973=DIRECTION('ref_axis',(1.,0.,0.));
#4974=DIRECTION('center_axis',(0.,1.,0.));
#4975=DIRECTION('ref_axis',(1.,0.,0.));
#4976=DIRECTION('center_axis',(0.,1.,0.));
#4977=DIRECTION('ref_axis',(1.,0.,0.));
#4978=DIRECTION('center_axis',(0.,1.,0.));
#4979=DIRECTION('ref_axis',(1.,0.,0.));
#4980=DIRECTION('',(0.,1.,0.));
#4981=DIRECTION('center_axis',(0.,1.,0.));
#4982=DIRECTION('ref_axis',(1.,0.,0.));
#4983=DIRECTION('center_axis',(0.,1.,0.));
#4984=DIRECTION('ref_axis',(1.,0.,0.));
#4985=DIRECTION('center_axis',(0.,1.,0.));
#4986=DIRECTION('ref_axis',(1.,0.,0.));
#4987=DIRECTION('center_axis',(0.,1.,0.));
#4988=DIRECTION('ref_axis',(1.,0.,0.));
#4989=DIRECTION('',(0.,1.,0.));
#4990=DIRECTION('center_axis',(0.,1.,0.));
#4991=DIRECTION('ref_axis',(1.,0.,0.));
#4992=DIRECTION('center_axis',(0.,1.,0.));
#4993=DIRECTION('ref_axis',(1.,0.,0.));
#4994=DIRECTION('center_axis',(0.,1.,0.));
#4995=DIRECTION('ref_axis',(1.,0.,0.));
#4996=DIRECTION('center_axis',(0.,1.,0.));
#4997=DIRECTION('ref_axis',(1.,0.,0.));
#4998=DIRECTION('',(0.,1.,0.));
#4999=DIRECTION('center_axis',(0.,1.,0.));
#5000=DIRECTION('ref_axis',(1.,0.,0.));
#5001=DIRECTION('center_axis',(0.,1.,0.));
#5002=DIRECTION('ref_axis',(1.,0.,0.));
#5003=DIRECTION('center_axis',(0.,1.,0.));
#5004=DIRECTION('ref_axis',(1.,0.,0.));
#5005=DIRECTION('center_axis',(0.,1.,0.));
#5006=DIRECTION('ref_axis',(1.,0.,0.));
#5007=DIRECTION('',(0.,1.,0.));
#5008=DIRECTION('center_axis',(0.,1.,0.));
#5009=DIRECTION('ref_axis',(1.,0.,0.));
#5010=DIRECTION('center_axis',(0.,1.,0.));
#5011=DIRECTION('ref_axis',(1.,0.,0.));
#5012=DIRECTION('center_axis',(0.,0.,1.));
#5013=DIRECTION('ref_axis',(1.,0.,0.));
#5014=DIRECTION('center_axis',(0.,0.,1.));
#5015=DIRECTION('ref_axis',(1.,0.,0.));
#5016=DIRECTION('',(0.,0.,1.));
#5017=DIRECTION('center_axis',(0.,0.,-1.));
#5018=DIRECTION('ref_axis',(1.,0.,0.));
#5019=DIRECTION('center_axis',(0.,0.,1.));
#5020=DIRECTION('ref_axis',(1.,0.,0.));
#5021=DIRECTION('center_axis',(0.,0.,1.));
#5022=DIRECTION('ref_axis',(1.,0.,0.));
#5023=DIRECTION('',(0.,0.,1.));
#5024=DIRECTION('center_axis',(0.,0.,-1.));
#5025=DIRECTION('ref_axis',(1.,0.,0.));
#5026=DIRECTION('center_axis',(0.,0.,1.));
#5027=DIRECTION('ref_axis',(1.,0.,0.));
#5028=DIRECTION('center_axis',(0.,0.,1.));
#5029=DIRECTION('ref_axis',(1.,0.,0.));
#5030=DIRECTION('',(0.,0.,1.));
#5031=DIRECTION('center_axis',(0.,0.,-1.));
#5032=DIRECTION('ref_axis',(1.,0.,0.));
#5033=DIRECTION('center_axis',(0.,0.,1.));
#5034=DIRECTION('ref_axis',(1.,0.,0.));
#5035=DIRECTION('center_axis',(0.,0.,1.));
#5036=DIRECTION('ref_axis',(1.,0.,0.));
#5037=DIRECTION('',(0.,0.,1.));
#5038=DIRECTION('center_axis',(0.,0.,-1.));
#5039=DIRECTION('ref_axis',(1.,0.,0.));
#5040=DIRECTION('center_axis',(0.,1.,0.));
#5041=DIRECTION('ref_axis',(0.,0.,1.));
#5042=DIRECTION('center_axis',(0.,1.,0.));
#5043=DIRECTION('ref_axis',(1.,0.,0.));
#5044=DIRECTION('',(1.,0.,0.));
#5045=DIRECTION('',(0.,0.,-1.));
#5046=DIRECTION('',(-1.,0.,0.));
#5047=DIRECTION('center_axis',(0.,1.,0.));
#5048=DIRECTION('ref_axis',(0.,0.,1.));
#5049=DIRECTION('center_axis',(0.,1.,0.));
#5050=DIRECTION('ref_axis',(1.,0.,0.));
#5051=DIRECTION('',(-1.,0.,0.));
#5052=DIRECTION('',(0.,0.,1.));
#5053=DIRECTION('',(1.,0.,0.));
#5054=DIRECTION('center_axis',(0.,1.,0.));
#5055=DIRECTION('ref_axis',(1.,0.,0.));
#5056=DIRECTION('center_axis',(0.,-1.,0.));
#5057=DIRECTION('ref_axis',(1.,0.,0.));
#5058=DIRECTION('',(1.,0.,0.));
#5059=DIRECTION('',(0.,0.,1.));
#5060=DIRECTION('',(-1.,0.,0.));
#5061=DIRECTION('center_axis',(0.,1.,0.));
#5062=DIRECTION('ref_axis',(1.,0.,0.));
#5063=DIRECTION('center_axis',(0.,-1.,0.));
#5064=DIRECTION('ref_axis',(1.,0.,0.));
#5065=DIRECTION('',(-1.,0.,0.));
#5066=DIRECTION('',(0.,0.,-1.));
#5067=DIRECTION('',(1.,0.,0.));
#5068=DIRECTION('center_axis',(0.,0.,1.));
#5069=DIRECTION('ref_axis',(1.,0.,0.));
#5070=DIRECTION('',(0.,1.,0.));
#5071=DIRECTION('',(0.,1.,0.));
#5072=DIRECTION('center_axis',(0.,0.,1.));
#5073=DIRECTION('ref_axis',(1.,0.,0.));
#5074=DIRECTION('',(0.,-1.,0.));
#5075=DIRECTION('',(0.,1.,0.));
#5076=DIRECTION('center_axis',(-1.,0.,0.));
#5077=DIRECTION('ref_axis',(0.,0.,1.));
#5078=DIRECTION('',(0.,1.,0.));
#5079=DIRECTION('center_axis',(0.,0.,-1.));
#5080=DIRECTION('ref_axis',(-1.,0.,0.));
#5081=DIRECTION('',(0.,1.,0.));
#5082=DIRECTION('center_axis',(1.,0.,0.));
#5083=DIRECTION('ref_axis',(0.,0.,-1.));
#5084=DIRECTION('center_axis',(0.,1.,0.));
#5085=DIRECTION('ref_axis',(0.,0.,1.));
#5086=DIRECTION('center_axis',(0.,1.,0.));
#5087=DIRECTION('ref_axis',(1.,0.,0.));
#5088=DIRECTION('',(1.,0.,0.));
#5089=DIRECTION('',(0.,0.,-1.));
#5090=DIRECTION('',(-1.,0.,0.));
#5091=DIRECTION('center_axis',(0.,1.,0.));
#5092=DIRECTION('ref_axis',(0.,0.,1.));
#5093=DIRECTION('center_axis',(0.,1.,0.));
#5094=DIRECTION('ref_axis',(1.,0.,0.));
#5095=DIRECTION('',(-1.,0.,0.));
#5096=DIRECTION('',(0.,0.,1.));
#5097=DIRECTION('',(1.,0.,0.));
#5098=DIRECTION('center_axis',(0.,1.,0.));
#5099=DIRECTION('ref_axis',(1.,0.,0.));
#5100=DIRECTION('center_axis',(0.,-1.,0.));
#5101=DIRECTION('ref_axis',(1.,0.,0.));
#5102=DIRECTION('',(1.,0.,0.));
#5103=DIRECTION('',(0.,0.,1.));
#5104=DIRECTION('',(-1.,0.,0.));
#5105=DIRECTION('center_axis',(0.,1.,0.));
#5106=DIRECTION('ref_axis',(1.,0.,0.));
#5107=DIRECTION('center_axis',(0.,-1.,0.));
#5108=DIRECTION('ref_axis',(1.,0.,0.));
#5109=DIRECTION('',(-1.,0.,0.));
#5110=DIRECTION('',(0.,0.,-1.));
#5111=DIRECTION('',(1.,0.,0.));
#5112=DIRECTION('center_axis',(0.,0.,1.));
#5113=DIRECTION('ref_axis',(1.,0.,0.));
#5114=DIRECTION('',(0.,1.,0.));
#5115=DIRECTION('',(0.,1.,0.));
#5116=DIRECTION('center_axis',(0.,0.,1.));
#5117=DIRECTION('ref_axis',(1.,0.,0.));
#5118=DIRECTION('',(0.,-1.,0.));
#5119=DIRECTION('',(0.,1.,0.));
#5120=DIRECTION('center_axis',(-1.,0.,0.));
#5121=DIRECTION('ref_axis',(0.,0.,1.));
#5122=DIRECTION('',(0.,1.,0.));
#5123=DIRECTION('center_axis',(0.,0.,-1.));
#5124=DIRECTION('ref_axis',(-1.,0.,0.));
#5125=DIRECTION('',(0.,1.,0.));
#5126=DIRECTION('center_axis',(1.,0.,0.));
#5127=DIRECTION('ref_axis',(0.,0.,-1.));
#5128=DIRECTION('center_axis',(0.,1.,0.));
#5129=DIRECTION('ref_axis',(1.,0.,0.));
#5130=DIRECTION('center_axis',(0.,-1.,0.));
#5131=DIRECTION('ref_axis',(1.,0.,0.));
#5132=DIRECTION('',(0.,-1.,0.));
#5133=DIRECTION('center_axis',(0.,-1.,0.));
#5134=DIRECTION('ref_axis',(1.,0.,0.));
#5135=DIRECTION('center_axis',(0.,1.,0.));
#5136=DIRECTION('ref_axis',(1.,0.,0.));
#5137=DIRECTION('center_axis',(0.,1.,0.));
#5138=DIRECTION('ref_axis',(1.,0.,0.));
#5139=DIRECTION('',(0.,-1.,0.));
#5140=DIRECTION('center_axis',(0.,1.,0.));
#5141=DIRECTION('ref_axis',(1.,0.,0.));
#5142=DIRECTION('center_axis',(0.,1.,0.));
#5143=DIRECTION('ref_axis',(1.,0.,0.));
#5144=DIRECTION('center_axis',(0.,1.,0.));
#5145=DIRECTION('ref_axis',(1.,0.,0.));
#6259=CARTESIAN_POINT('',(0.,0.,0.));
#6260=CARTESIAN_POINT('Origin',(-2.8,4.4,4.5));
#6261=CARTESIAN_POINT('',(-2.965,4.4,4.5));
#6262=CARTESIAN_POINT('Origin',(-2.8,4.4,4.5));
#6263=CARTESIAN_POINT('',(-2.965,6.,4.5));
#6264=CARTESIAN_POINT('',(-2.965,4.4,4.5));
#6265=CARTESIAN_POINT('Origin',(-2.8,6.,4.5));
#6266=CARTESIAN_POINT('Origin',(-2.8,4.4,4.5));
#6267=CARTESIAN_POINT('Origin',(1.71450551880629E-16,4.4,7.3));
#6268=CARTESIAN_POINT('',(-0.165,4.4,7.3));
#6269=CARTESIAN_POINT('Origin',(1.71450551880629E-16,4.4,7.3));
#6270=CARTESIAN_POINT('',(-0.165,6.,7.3));
#6271=CARTESIAN_POINT('',(-0.165,4.4,7.3));
#6272=CARTESIAN_POINT('Origin',(1.71450551880629E-16,6.,7.3));
#6273=CARTESIAN_POINT('Origin',(1.66533453693773E-16,4.4,7.3));
#6274=CARTESIAN_POINT('Origin',(2.8,4.4,4.5));
#6275=CARTESIAN_POINT('',(2.635,4.4,4.5));
#6276=CARTESIAN_POINT('Origin',(2.8,4.4,4.5));
#6277=CARTESIAN_POINT('',(2.635,6.,4.5));
#6278=CARTESIAN_POINT('',(2.635,4.4,4.5));
#6279=CARTESIAN_POINT('Origin',(2.8,6.,4.5));
#6280=CARTESIAN_POINT('Origin',(2.8,4.4,4.5));
#6281=CARTESIAN_POINT('Origin',(-5.14351655641888E-16,4.4,1.7));
#6282=CARTESIAN_POINT('',(-0.165000000000001,4.4,1.7));
#6283=CARTESIAN_POINT('Origin',(-5.14351655641888E-16,4.4,1.7));
#6284=CARTESIAN_POINT('',(-0.165000000000001,6.,1.7));
#6285=CARTESIAN_POINT('',(-0.165000000000001,4.4,1.7));
#6286=CARTESIAN_POINT('Origin',(-5.14351655641888E-16,6.,1.7));
#6287=CARTESIAN_POINT('Origin',(-5.27355936696949E-16,4.4,1.7));
#6288=CARTESIAN_POINT('Origin',(-2.8,-0.1,4.5));
#6289=CARTESIAN_POINT('',(-2.965,0.,4.5));
#6290=CARTESIAN_POINT('Origin',(-2.8,0.,4.5));
#6291=CARTESIAN_POINT('',(-2.965,1.6,4.5));
#6292=CARTESIAN_POINT('',(-2.965,-0.1,4.5));
#6293=CARTESIAN_POINT('Origin',(-2.8,1.6,4.5));
#6294=CARTESIAN_POINT('Origin',(-2.8,1.6,4.5));
#6295=CARTESIAN_POINT('Origin',(1.71450551880629E-16,-0.1,7.3));
#6296=CARTESIAN_POINT('',(-0.165,0.,7.3));
#6297=CARTESIAN_POINT('Origin',(1.71450551880629E-16,0.,7.3));
#6298=CARTESIAN_POINT('',(-0.165,1.6,7.3));
#6299=CARTESIAN_POINT('',(-0.165,-0.1,7.3));
#6300=CARTESIAN_POINT('Origin',(1.71450551880629E-16,1.6,7.3));
#6301=CARTESIAN_POINT('Origin',(1.66533453693773E-16,1.6,7.3));
#6302=CARTESIAN_POINT('Origin',(2.8,-0.1,4.5));
#6303=CARTESIAN_POINT('',(2.635,0.,4.5));
#6304=CARTESIAN_POINT('Origin',(2.8,0.,4.5));
#6305=CARTESIAN_POINT('',(2.635,1.6,4.5));
#6306=CARTESIAN_POINT('',(2.635,-0.1,4.5));
#6307=CARTESIAN_POINT('Origin',(2.8,1.6,4.5));
#6308=CARTESIAN_POINT('Origin',(2.8,1.6,4.5));
#6309=CARTESIAN_POINT('Origin',(-5.14351655641888E-16,-0.1,1.7));
#6310=CARTESIAN_POINT('',(-0.165000000000001,0.,1.7));
#6311=CARTESIAN_POINT('Origin',(-5.14351655641888E-16,0.,1.7));
#6312=CARTESIAN_POINT('',(-0.165000000000001,1.6,1.7));
#6313=CARTESIAN_POINT('',(-0.165000000000001,-0.1,1.7));
#6314=CARTESIAN_POINT('Origin',(-5.14351655641888E-16,1.6,1.7));
#6315=CARTESIAN_POINT('Origin',(-5.27355936696949E-16,1.6,1.7));
#6316=CARTESIAN_POINT('Origin',(3.8,1.,0.9));
#6317=CARTESIAN_POINT('',(3.47,1.,1.));
#6318=CARTESIAN_POINT('Origin',(3.8,1.,1.));
#6319=CARTESIAN_POINT('',(3.47,1.,2.5));
#6320=CARTESIAN_POINT('',(3.47,1.,0.9));
#6321=CARTESIAN_POINT('Origin',(3.8,1.,2.5));
#6322=CARTESIAN_POINT('Origin',(-3.8,5.,0.9));
#6323=CARTESIAN_POINT('',(-4.13,5.,1.));
#6324=CARTESIAN_POINT('Origin',(-3.8,5.,1.));
#6325=CARTESIAN_POINT('',(-4.13,5.,2.5));
#6326=CARTESIAN_POINT('',(-4.13,5.,0.9));
#6327=CARTESIAN_POINT('Origin',(-3.8,5.,2.5));
#6328=CARTESIAN_POINT('Origin',(-3.8,1.,0.9));
#6329=CARTESIAN_POINT('',(-4.13,1.,1.));
#6330=CARTESIAN_POINT('Origin',(-3.8,1.,1.));
#6331=CARTESIAN_POINT('',(-4.13,1.,2.5));
#6332=CARTESIAN_POINT('',(-4.13,1.,0.9));
#6333=CARTESIAN_POINT('Origin',(-3.8,1.,2.5));
#6334=CARTESIAN_POINT('Origin',(3.8,5.,0.9));
#6335=CARTESIAN_POINT('',(3.47,5.,1.));
#6336=CARTESIAN_POINT('Origin',(3.8,5.,1.));
#6337=CARTESIAN_POINT('',(3.47,5.,2.5));
#6338=CARTESIAN_POINT('',(3.47,5.,0.9));
#6339=CARTESIAN_POINT('Origin',(3.8,5.,2.5));
#6340=CARTESIAN_POINT('Origin',(0.,5.5,1.75));
#6341=CARTESIAN_POINT('',(2.87228132326901,5.5,2.5));
#6342=CARTESIAN_POINT('',(0.,5.5,1.));
#6343=CARTESIAN_POINT('Origin',(0.,5.5,4.5));
#6344=CARTESIAN_POINT('',(4.5,5.5,2.5));
#6345=CARTESIAN_POINT('',(4.5,5.5,2.5));
#6346=CARTESIAN_POINT('',(4.5,5.5,1.));
#6347=CARTESIAN_POINT('',(4.5,5.5,1.));
#6348=CARTESIAN_POINT('',(-4.5,5.5,1.));
#6349=CARTESIAN_POINT('Origin',(0.,5.5,1.75));
#6350=CARTESIAN_POINT('',(-2.87228132326901,5.5,2.5));
#6351=CARTESIAN_POINT('Origin',(0.,5.5,4.5));
#6352=CARTESIAN_POINT('',(-4.5,5.5,1.));
#6353=CARTESIAN_POINT('',(-4.5,5.5,1.));
#6354=CARTESIAN_POINT('',(-4.5,5.5,2.5));
#6355=CARTESIAN_POINT('',(-4.5,5.5,2.5));
#6356=CARTESIAN_POINT('',(4.5,5.5,2.5));
#6357=CARTESIAN_POINT('Origin',(0.,4.5,1.75));
#6358=CARTESIAN_POINT('',(0.,4.5,1.));
#6359=CARTESIAN_POINT('',(2.87228132326901,4.5,2.5));
#6360=CARTESIAN_POINT('Origin',(0.,4.5,4.5));
#6361=CARTESIAN_POINT('',(4.5,4.5,1.));
#6362=CARTESIAN_POINT('',(-4.5,4.5,1.));
#6363=CARTESIAN_POINT('',(4.5,4.5,2.5));
#6364=CARTESIAN_POINT('',(4.5,4.5,1.));
#6365=CARTESIAN_POINT('',(4.5,4.5,2.5));
#6366=CARTESIAN_POINT('Origin',(0.,4.5,1.75));
#6367=CARTESIAN_POINT('',(-2.87228132326901,4.5,2.5));
#6368=CARTESIAN_POINT('Origin',(0.,4.5,4.5));
#6369=CARTESIAN_POINT('',(-4.5,4.5,2.5));
#6370=CARTESIAN_POINT('',(4.5,4.5,2.5));
#6371=CARTESIAN_POINT('',(-4.5,4.5,1.));
#6372=CARTESIAN_POINT('',(-4.5,4.5,2.5));
#6373=CARTESIAN_POINT('',(-4.5,4.5,1.));
#6374=CARTESIAN_POINT('Origin',(-4.5,4.5,2.5));
#6375=CARTESIAN_POINT('',(2.87228132326901,0.,2.5));
#6376=CARTESIAN_POINT('',(4.5,4.5,2.5));
#6377=CARTESIAN_POINT('Origin',(-4.5,4.5,2.5));
#6378=CARTESIAN_POINT('',(-2.87228132326901,0.,2.5));
#6379=CARTESIAN_POINT('',(-4.5,4.5,2.5));
#6380=CARTESIAN_POINT('Origin',(-4.5,4.5,1.));
#6381=CARTESIAN_POINT('',(-4.5,4.5,1.));
#6382=CARTESIAN_POINT('Origin',(4.5,4.5,1.));
#6383=CARTESIAN_POINT('',(4.5,4.5,1.));
#6384=CARTESIAN_POINT('Origin',(4.5,4.5,2.5));
#6385=CARTESIAN_POINT('Origin',(0.,1.5,1.75));
#6386=CARTESIAN_POINT('',(2.87228132326901,1.5,2.5));
#6387=CARTESIAN_POINT('',(0.,1.5,1.));
#6388=CARTESIAN_POINT('Origin',(0.,1.5,4.5));
#6389=CARTESIAN_POINT('',(4.5,1.5,2.5));
#6390=CARTESIAN_POINT('',(4.5,1.5,2.5));
#6391=CARTESIAN_POINT('',(4.5,1.5,1.));
#6392=CARTESIAN_POINT('',(4.5,1.5,1.));
#6393=CARTESIAN_POINT('',(-4.5,1.5,1.));
#6394=CARTESIAN_POINT('Origin',(0.,1.5,1.75));
#6395=CARTESIAN_POINT('',(-2.87228132326901,1.5,2.5));
#6396=CARTESIAN_POINT('Origin',(0.,1.5,4.5));
#6397=CARTESIAN_POINT('',(-4.5,1.5,1.));
#6398=CARTESIAN_POINT('',(-4.5,1.5,1.));
#6399=CARTESIAN_POINT('',(-4.5,1.5,2.5));
#6400=CARTESIAN_POINT('',(-4.5,1.5,2.5));
#6401=CARTESIAN_POINT('',(4.5,1.5,2.5));
#6402=CARTESIAN_POINT('Origin',(0.,0.5,1.75));
#6403=CARTESIAN_POINT('',(0.,0.5,1.));
#6404=CARTESIAN_POINT('',(2.87228132326901,0.5,2.5));
#6405=CARTESIAN_POINT('Origin',(0.,0.5,4.5));
#6406=CARTESIAN_POINT('',(4.5,0.5,1.));
#6407=CARTESIAN_POINT('',(-4.5,0.5,1.));
#6408=CARTESIAN_POINT('',(4.5,0.5,2.5));
#6409=CARTESIAN_POINT('',(4.5,0.5,1.));
#6410=CARTESIAN_POINT('',(4.5,0.5,2.5));
#6411=CARTESIAN_POINT('Origin',(0.,0.5,1.75));
#6412=CARTESIAN_POINT('',(-2.87228132326901,0.5,2.5));
#6413=CARTESIAN_POINT('Origin',(0.,0.5,4.5));
#6414=CARTESIAN_POINT('',(-4.5,0.5,2.5));
#6415=CARTESIAN_POINT('',(4.5,0.5,2.5));
#6416=CARTESIAN_POINT('',(-4.5,0.5,1.));
#6417=CARTESIAN_POINT('',(-4.5,0.5,2.5));
#6418=CARTESIAN_POINT('',(-4.5,0.5,1.));
#6419=CARTESIAN_POINT('Origin',(-4.5,0.5,2.5));
#6420=CARTESIAN_POINT('',(2.87228132326901,0.,2.5));
#6421=CARTESIAN_POINT('',(4.5,0.5,2.5));
#6422=CARTESIAN_POINT('Origin',(-4.5,0.5,2.5));
#6423=CARTESIAN_POINT('',(-2.87228132326901,0.,2.5));
#6424=CARTESIAN_POINT('',(-4.5,0.5,2.5));
#6425=CARTESIAN_POINT('Origin',(-4.5,0.5,1.));
#6426=CARTESIAN_POINT('',(-4.5,0.5,1.));
#6427=CARTESIAN_POINT('Origin',(4.5,0.5,1.));
#6428=CARTESIAN_POINT('',(4.5,0.5,1.));
#6429=CARTESIAN_POINT('Origin',(4.5,0.5,2.5));
#6430=CARTESIAN_POINT('Origin',(0.,0.,4.5));
#6431=CARTESIAN_POINT('',(-2.35,6.,4.5));
#6432=CARTESIAN_POINT('Origin',(0.,6.,4.5));
#6433=CARTESIAN_POINT('',(-2.35,0.,4.5));
#6434=CARTESIAN_POINT('',(-2.35,0.,4.5));
#6435=CARTESIAN_POINT('Origin',(0.,0.,4.5));
#6436=CARTESIAN_POINT('Origin',(0.,0.,4.5));
#6437=CARTESIAN_POINT('',(-3.5,6.,4.5));
#6438=CARTESIAN_POINT('Origin',(0.,6.,4.5));
#6439=CARTESIAN_POINT('',(-3.5,0.,4.5));
#6440=CARTESIAN_POINT('',(-3.5,0.,4.5));
#6441=CARTESIAN_POINT('Origin',(0.,0.,4.5));
#6442=CARTESIAN_POINT('Origin',(0.,6.,4.5));
#6443=CARTESIAN_POINT('Origin',(0.,0.,4.5));
#7823=UNCERTAINTY_MEASURE_WITH_UNIT(LENGTH_MEASURE(0.001),#7872,
'DISTANCE_ACCURACY_VALUE',
'Maximum model space distance between geometric entities at asserted c
onnectivities');
#7845=UNCERTAINTY_MEASURE_WITH_UNIT(LENGTH_MEASURE(0.001),#7872,
'DISTANCE_ACCURACY_VALUE',
'Maximum model space distance between geometric entities at asserted c
onnectivities');
#7849=(
GEOMETRIC_REPRESENTATION_CONTEXT(3)
GLOBAL_UNCERTAINTY_ASSIGNED_CONTEXT((#7823))
GLOBAL_UNIT_ASSIGNED_CONTEXT((#7872,#7874,#7875))
REPRESENTATION_CONTEXT('','3D')
);
#7871=(
GEOMETRIC_REPRESENTATION_CONTEXT(3)
GLOBAL_UNCERTAINTY_ASSIGNED_CONTEXT((#7845))
GLOBAL_UNIT_ASSIGNED_CONTEXT((#7872,#7874,#7875))
REPRESENTATION_CONTEXT('','3D')
);
#7872=(
LENGTH_UNIT()
NAMED_UNIT(*)
SI_UNIT(.CENTI.,.METRE.)
);
#7874=(
NAMED_UNIT(*)
PLANE_ANGLE_UNIT()
SI_UNIT($,.RADIAN.)
);
#7875=(
NAMED_UNIT(*)
SI_UNIT($,.STERADIAN.)
SOLID_ANGLE_UNIT()
);
#7879=SHAPE_DEFINITION_REPRESENTATION(#7904,#7965);
#7904=PRODUCT_DEFINITION_SHAPE('',$,#7991);
#7965=SHAPE_REPRESENTATION('',(#4369),#7849);
#7987=PRODUCT_DEFINITION_CONTEXT('part definition',#8064,'design');
#7991=PRODUCT_DEFINITION('Housing','Housing',#8016,#7987);
#8016=PRODUCT_DEFINITION_FORMATION('',$,#8069);
#8064=APPLICATION_CONTEXT(
'Core Data for Automotive Mechanical Design Process');
#8065=PRODUCT_CONTEXT('part definition',#8064,'mechanical');
#8069=PRODUCT('Housing','Housing','Housing',(#8065));
#8126=COLOUR_RGB('Dark Blue',0.08,0.2,0.34);
#8127=FILL_AREA_STYLE_COLOUR('',#8126);
#8128=FILL_AREA_STYLE('',(#8127));
#8129=SURFACE_STYLE_FILL_AREA(#8128);
#8130=SURFACE_SIDE_STYLE('',(#8129));
#8131=SURFACE_STYLE_USAGE(.BOTH.,#8130);
#8132=PRESENTATION_STYLE_ASSIGNMENT((#8131));
ENDSEC;
END-ISO-10303-21;
